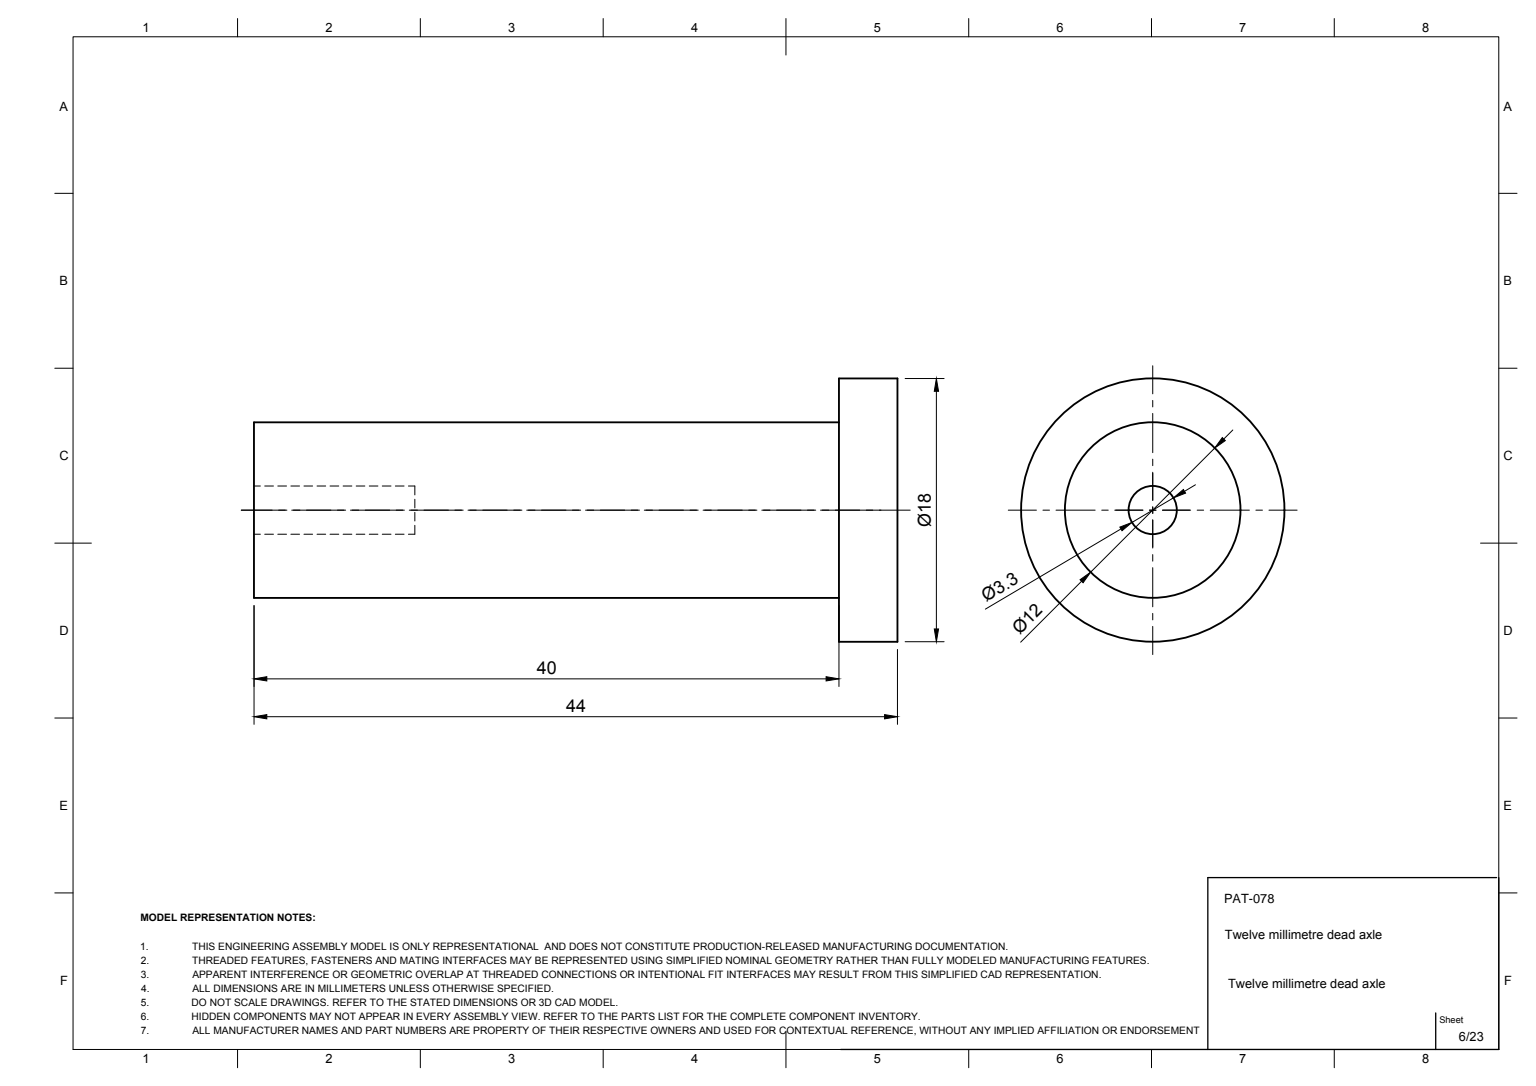
ISO-10303-21;
HEADER;
/* Generated by software containing ST-Developer
 * from STEP Tools, Inc. (www.steptools.com) 
 */

FILE_DESCRIPTION(
/* description */ ('Pedal-braked fixed caster'),
/* implementation_level */ '2;1');

FILE_NAME(
/* name */ 'Twelve millimetre dead axle.step',
/* time_stamp */ '2026-10-28T03:26:52-07:00',
/* author */ (''),
/* organization */ (''),
/* preprocessor_version */ 'ST-DEVELOPER v20.2',
/* originating_system */ 'Autodesk Translation Framework v15.17.0.0',
/* authorisation */ '');

FILE_SCHEMA (('AUTOMOTIVE_DESIGN { 1 0 10303 214 3 1 1 }'));
ENDSEC;

DATA;
#10=MECHANICAL_DESIGN_GEOMETRIC_PRESENTATION_REPRESENTATION('',(#207),#5734);
#173=SHAPE_REPRESENTATION_RELATIONSHIP('SRR','None',#5811,#190);
#190=ADVANCED_BREP_SHAPE_REPRESENTATION('',(#231),#5715);
#207=STYLED_ITEM('',(#5984),#231);
#231=MANIFOLD_SOLID_BREP('Body1',#2988);
#261=CYLINDRICAL_SURFACE('',#3262,0.165);
#262=CYLINDRICAL_SURFACE('',#3269,0.9);
#263=CYLINDRICAL_SURFACE('',#3272,0.6);
#311=FACE_BOUND('',#715,.T.);
#312=FACE_BOUND('',#720,.T.);
#356=CIRCLE('',#3263,0.165);
#357=CIRCLE('',#3264,0.165);
#358=CIRCLE('',#3267,0.9);
#359=CIRCLE('',#3268,0.6);
#360=CIRCLE('',#3270,0.9);
#361=CIRCLE('',#3273,0.6);
#518=FACE_OUTER_BOUND('',#712,.T.);
#519=FACE_OUTER_BOUND('',#713,.T.);
#520=FACE_OUTER_BOUND('',#714,.T.);
#521=FACE_OUTER_BOUND('',#716,.T.);
#522=FACE_OUTER_BOUND('',#717,.T.);
#523=FACE_OUTER_BOUND('',#718,.T.);
#524=FACE_OUTER_BOUND('',#719,.T.);
#712=EDGE_LOOP('',(#2168,#2169,#2170,#2171));
#713=EDGE_LOOP('',(#2172));
#714=EDGE_LOOP('',(#2173));
#715=EDGE_LOOP('',(#2174));
#716=EDGE_LOOP('',(#2175,#2176,#2177,#2178));
#717=EDGE_LOOP('',(#2179));
#718=EDGE_LOOP('',(#2180,#2181,#2182,#2183));
#719=EDGE_LOOP('',(#2184));
#720=EDGE_LOOP('',(#2185));
#975=LINE('',#4735,#1187);
#976=LINE('',#4745,#1188);
#977=LINE('',#4751,#1189);
#1187=VECTOR('',#3787,0.165);
#1188=VECTOR('',#3800,0.9);
#1189=VECTOR('',#3809,0.6);
#1377=VERTEX_POINT('',#4732);
#1378=VERTEX_POINT('',#4734);
#1379=VERTEX_POINT('',#4739);
#1380=VERTEX_POINT('',#4741);
#1381=VERTEX_POINT('',#4744);
#1382=VERTEX_POINT('',#4749);
#1674=EDGE_CURVE('',#1377,#1377,#356,.T.);
#1675=EDGE_CURVE('',#1377,#1378,#975,.T.);
#1676=EDGE_CURVE('',#1378,#1378,#357,.T.);
#1677=EDGE_CURVE('',#1379,#1379,#358,.T.);
#1678=EDGE_CURVE('',#1380,#1380,#359,.T.);
#1679=EDGE_CURVE('',#1379,#1381,#976,.T.);
#1680=EDGE_CURVE('',#1381,#1381,#360,.T.);
#1681=EDGE_CURVE('',#1382,#1382,#361,.T.);
#1682=EDGE_CURVE('',#1382,#1380,#977,.T.);
#2168=ORIENTED_EDGE('',*,*,#1674,.F.);
#2169=ORIENTED_EDGE('',*,*,#1675,.T.);
#2170=ORIENTED_EDGE('',*,*,#1676,.F.);
#2171=ORIENTED_EDGE('',*,*,#1675,.F.);
#2172=ORIENTED_EDGE('',*,*,#1674,.T.);
#2173=ORIENTED_EDGE('',*,*,#1677,.T.);
#2174=ORIENTED_EDGE('',*,*,#1678,.F.);
#2175=ORIENTED_EDGE('',*,*,#1677,.F.);
#2176=ORIENTED_EDGE('',*,*,#1679,.T.);
#2177=ORIENTED_EDGE('',*,*,#1680,.T.);
#2178=ORIENTED_EDGE('',*,*,#1679,.F.);
#2179=ORIENTED_EDGE('',*,*,#1680,.F.);
#2180=ORIENTED_EDGE('',*,*,#1681,.F.);
#2181=ORIENTED_EDGE('',*,*,#1682,.T.);
#2182=ORIENTED_EDGE('',*,*,#1678,.T.);
#2183=ORIENTED_EDGE('',*,*,#1682,.F.);
#2184=ORIENTED_EDGE('',*,*,#1681,.T.);
#2185=ORIENTED_EDGE('',*,*,#1676,.T.);
#2734=PLANE('',#3265);
#2735=PLANE('',#3266);
#2736=PLANE('',#3271);
#2737=PLANE('',#3274);
#2851=ADVANCED_FACE('',(#518),#261,.F.);
#2852=ADVANCED_FACE('',(#519),#2734,.T.);
#2853=ADVANCED_FACE('',(#520,#311),#2735,.T.);
#2854=ADVANCED_FACE('',(#521),#262,.T.);
#2855=ADVANCED_FACE('',(#522),#2736,.F.);
#2856=ADVANCED_FACE('',(#523),#263,.T.);
#2857=ADVANCED_FACE('',(#524,#312),#2737,.T.);
#2988=CLOSED_SHELL('',(#2851,#2852,#2853,#2854,#2855,#2856,#2857));
#3261=AXIS2_PLACEMENT_3D('',#4730,#3781,#3782);
#3262=AXIS2_PLACEMENT_3D('',#4731,#3783,#3784);
#3263=AXIS2_PLACEMENT_3D('',#4733,#3785,#3786);
#3264=AXIS2_PLACEMENT_3D('',#4736,#3788,#3789);
#3265=AXIS2_PLACEMENT_3D('',#4737,#3790,#3791);
#3266=AXIS2_PLACEMENT_3D('',#4738,#3792,#3793);
#3267=AXIS2_PLACEMENT_3D('',#4740,#3794,#3795);
#3268=AXIS2_PLACEMENT_3D('',#4742,#3796,#3797);
#3269=AXIS2_PLACEMENT_3D('',#4743,#3798,#3799);
#3270=AXIS2_PLACEMENT_3D('',#4746,#3801,#3802);
#3271=AXIS2_PLACEMENT_3D('',#4747,#3803,#3804);
#3272=AXIS2_PLACEMENT_3D('',#4748,#3805,#3806);
#3273=AXIS2_PLACEMENT_3D('',#4750,#3807,#3808);
#3274=AXIS2_PLACEMENT_3D('',#4752,#3810,#3811);
#3781=DIRECTION('axis',(0.,0.,1.));
#3782=DIRECTION('refdir',(1.,0.,0.));
#3783=DIRECTION('center_axis',(0.,1.,0.));
#3784=DIRECTION('ref_axis',(1.,0.,0.));
#3785=DIRECTION('center_axis',(0.,1.,0.));
#3786=DIRECTION('ref_axis',(1.,0.,0.));
#3787=DIRECTION('',(0.,1.,0.));
#3788=DIRECTION('center_axis',(0.,-1.,0.));
#3789=DIRECTION('ref_axis',(1.,0.,0.));
#3790=DIRECTION('center_axis',(0.,1.,0.));
#3791=DIRECTION('ref_axis',(1.,0.,0.));
#3792=DIRECTION('center_axis',(0.,1.,0.));
#3793=DIRECTION('ref_axis',(1.,0.,0.));
#3794=DIRECTION('center_axis',(0.,1.,0.));
#3795=DIRECTION('ref_axis',(1.,0.,0.));
#3796=DIRECTION('center_axis',(0.,1.,0.));
#3797=DIRECTION('ref_axis',(1.,0.,0.));
#3798=DIRECTION('center_axis',(0.,1.,0.));
#3799=DIRECTION('ref_axis',(1.,0.,0.));
#3800=DIRECTION('',(0.,-1.,0.));
#3801=DIRECTION('center_axis',(0.,1.,0.));
#3802=DIRECTION('ref_axis',(1.,0.,0.));
#3803=DIRECTION('center_axis',(0.,1.,0.));
#3804=DIRECTION('ref_axis',(1.,0.,0.));
#3805=DIRECTION('center_axis',(0.,1.,0.));
#3806=DIRECTION('ref_axis',(1.,0.,0.));
#3807=DIRECTION('center_axis',(0.,1.,0.));
#3808=DIRECTION('ref_axis',(1.,0.,0.));
#3809=DIRECTION('',(0.,-1.,0.));
#3810=DIRECTION('center_axis',(0.,1.,0.));
#3811=DIRECTION('ref_axis',(1.,0.,0.));
#4730=CARTESIAN_POINT('',(0.,0.,0.));
#4731=CARTESIAN_POINT('Origin',(0.,0.9,3.5));
#4732=CARTESIAN_POINT('',(-0.165,0.9,3.5));
#4733=CARTESIAN_POINT('Origin',(0.,0.9,3.5));
#4734=CARTESIAN_POINT('',(-0.165,2.,3.5));
#4735=CARTESIAN_POINT('',(-0.165,0.9,3.5));
#4736=CARTESIAN_POINT('Origin',(0.,2.,3.5));
#4737=CARTESIAN_POINT('Origin',(0.,0.9,3.5));
#4738=CARTESIAN_POINT('Origin',(0.,-2.,3.5));
#4739=CARTESIAN_POINT('',(-0.9,-2.,3.5));
#4740=CARTESIAN_POINT('Origin',(0.,-2.,3.5));
#4741=CARTESIAN_POINT('',(-0.6,-2.,3.5));
#4742=CARTESIAN_POINT('Origin',(0.,-2.,3.5));
#4743=CARTESIAN_POINT('Origin',(0.,-2.4,3.5));
#4744=CARTESIAN_POINT('',(-0.9,-2.4,3.5));
#4745=CARTESIAN_POINT('',(-0.9,-2.4,3.5));
#4746=CARTESIAN_POINT('Origin',(0.,-2.4,3.5));
#4747=CARTESIAN_POINT('Origin',(0.,-2.4,3.5));
#4748=CARTESIAN_POINT('Origin',(0.,-2.,3.5));
#4749=CARTESIAN_POINT('',(-0.6,2.,3.5));
#4750=CARTESIAN_POINT('Origin',(0.,2.,3.5));
#4751=CARTESIAN_POINT('',(-0.6,-2.,3.5));
#4752=CARTESIAN_POINT('Origin',(0.,2.,3.5));
#5692=UNCERTAINTY_MEASURE_WITH_UNIT(LENGTH_MEASURE(0.001),#5735,
'DISTANCE_ACCURACY_VALUE',
'Maximum model space distance between geometric entities at asserted c
onnectivities');
#5711=UNCERTAINTY_MEASURE_WITH_UNIT(LENGTH_MEASURE(0.001),#5735,
'DISTANCE_ACCURACY_VALUE',
'Maximum model space distance between geometric entities at asserted c
onnectivities');
#5715=(
GEOMETRIC_REPRESENTATION_CONTEXT(3)
GLOBAL_UNCERTAINTY_ASSIGNED_CONTEXT((#5692))
GLOBAL_UNIT_ASSIGNED_CONTEXT((#5735,#5737,#5738))
REPRESENTATION_CONTEXT('','3D')
);
#5734=(
GEOMETRIC_REPRESENTATION_CONTEXT(3)
GLOBAL_UNCERTAINTY_ASSIGNED_CONTEXT((#5711))
GLOBAL_UNIT_ASSIGNED_CONTEXT((#5735,#5737,#5738))
REPRESENTATION_CONTEXT('','3D')
);
#5735=(
LENGTH_UNIT()
NAMED_UNIT(*)
SI_UNIT(.CENTI.,.METRE.)
);
#5737=(
NAMED_UNIT(*)
PLANE_ANGLE_UNIT()
SI_UNIT($,.RADIAN.)
);
#5738=(
NAMED_UNIT(*)
SI_UNIT($,.STERADIAN.)
SOLID_ANGLE_UNIT()
);
#5742=SHAPE_DEFINITION_REPRESENTATION(#5764,#5811);
#5764=PRODUCT_DEFINITION_SHAPE('',$,#5834);
#5811=SHAPE_REPRESENTATION('',(#3261),#5715);
#5830=PRODUCT_DEFINITION_CONTEXT('part definition',#5898,'design');
#5834=PRODUCT_DEFINITION('Twelve millimetre dead axle',
'Twelve millimetre dead axle',#5856,#5830);
#5856=PRODUCT_DEFINITION_FORMATION('',$,#5903);
#5898=APPLICATION_CONTEXT(
'Core Data for Automotive Mechanical Design Process');
#5899=PRODUCT_CONTEXT('part definition',#5898,'mechanical');
#5903=PRODUCT('Twelve millimetre dead axle',
'Twelve millimetre dead axle','Twelve millimetre dead axle',(#5899));
#5978=COLOUR_RGB('Grey',0.48,0.52,0.57);
#5979=FILL_AREA_STYLE_COLOUR('',#5978);
#5980=FILL_AREA_STYLE('',(#5979));
#5981=SURFACE_STYLE_FILL_AREA(#5980);
#5982=SURFACE_SIDE_STYLE('',(#5981));
#5983=SURFACE_STYLE_USAGE(.BOTH.,#5982);
#5984=PRESENTATION_STYLE_ASSIGNMENT((#5983));
ENDSEC;
END-ISO-10303-21;
